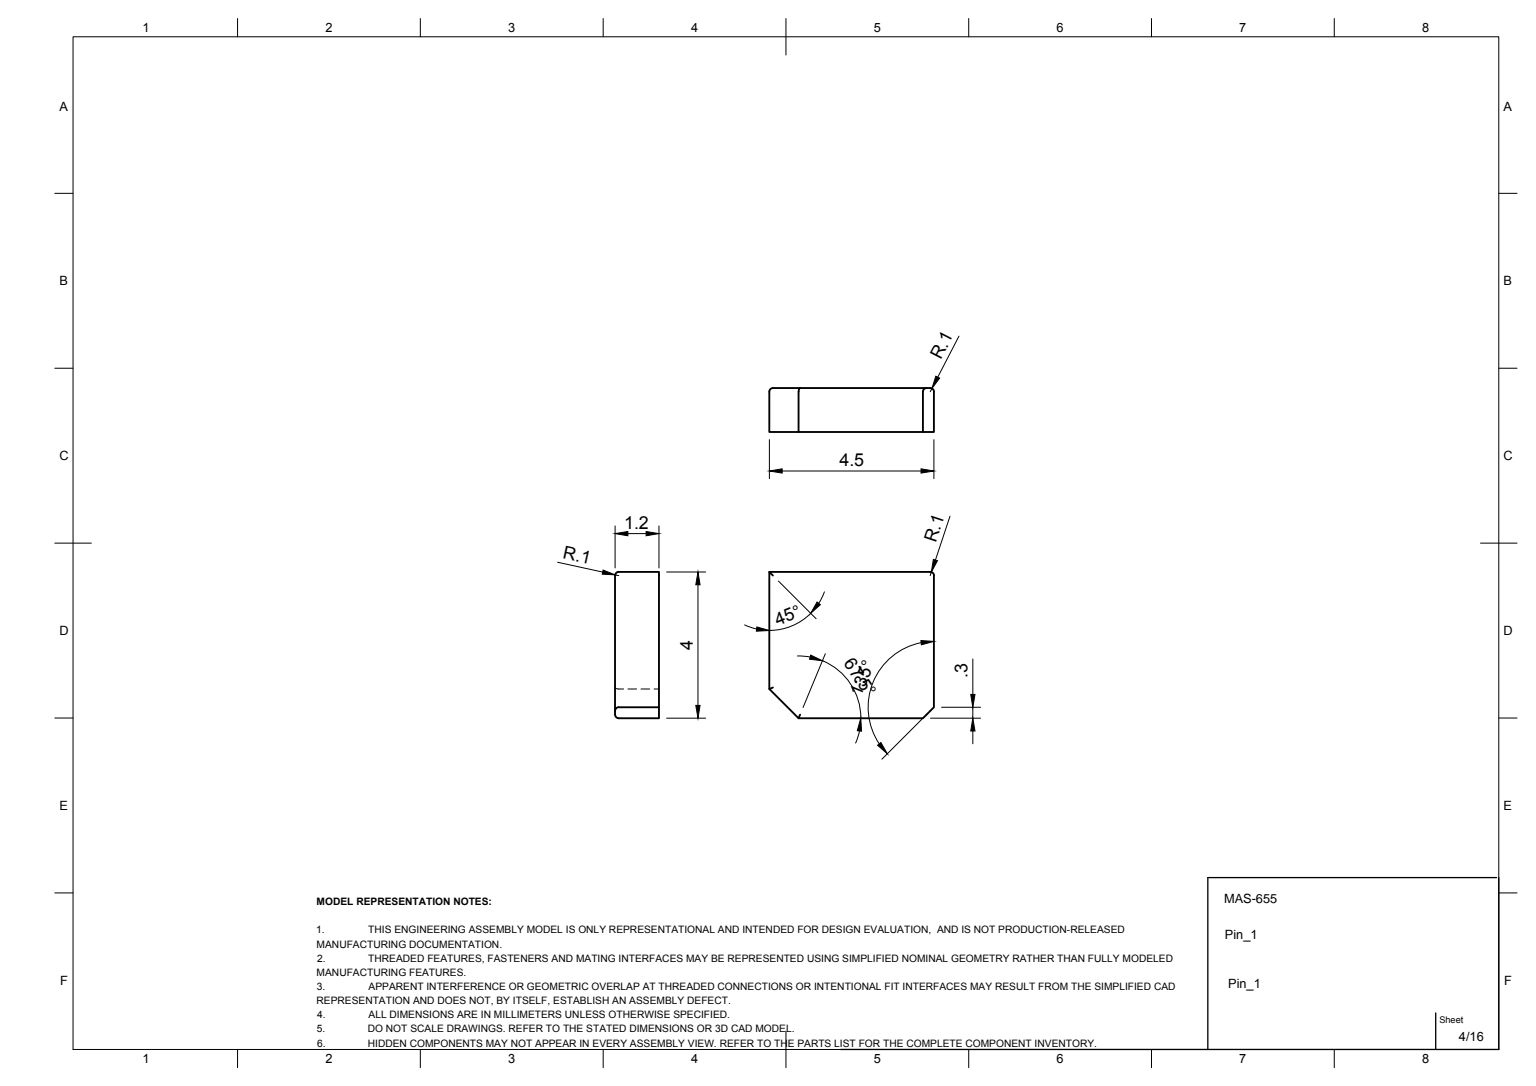
ISO-10303-21;
HEADER;
FILE_DESCRIPTION((''),'2;1');
FILE_NAME('Pin_1.step','2026-10-09T11:34:15-07:00',(''),(''),'','','');
FILE_SCHEMA (('AUTOMOTIVE_DESIGN { 1 0 10303 214 3 1 1 }'));
ENDSEC;
DATA;
#10=MECHANICAL_DESIGN_GEOMETRIC_PRESENTATION_REPRESENTATION('',(#631),#117170);
#264=ELLIPSE('',#51711,0.141421356237302,0.1) ;
#265=ELLIPSE('',#51712,0.108239220029239,0.1) ;
#266=ELLIPSE('',#51714,0.108239220029249,0.1) ;
#267=ELLIPSE('',#51716,0.141421356237297,0.1) ;
#268=ELLIPSE('',#51722,0.141421356237317,0.1) ;
#589=SHAPE_REPRESENTATION_RELATIONSHIP('SRR','None',#117244,#610) ;
#610=ADVANCED_BREP_SHAPE_REPRESENTATION('',(#652),#117152) ;
#631=STYLED_ITEM('',(#117355),#652) ;
#652=MANIFOLD_SOLID_BREP('Body1',#49060) ;
#2192=SPHERICAL_SURFACE('',#51717,0.100000000000016) ;
#2427=PLANE('',#51726) ;
#2428=PLANE('',#51727) ;
#2429=PLANE('',#51728) ;
#2430=PLANE('',#51729) ;
#2431=PLANE('',#51730) ;
#2432=PLANE('',#51731) ;
#2433=PLANE('',#51732) ;
#2434=PLANE('',#51733) ;
#4081=LINE('',#86546,#7295) ;
#4082=LINE('',#86550,#7296) ;
#4083=LINE('',#86554,#7297) ;
#4084=LINE('',#86557,#7298) ;
#4085=LINE('',#86560,#7299) ;
#4086=LINE('',#86563,#7300) ;
#4087=LINE('',#86575,#7301) ;
#4088=LINE('',#86576,#7302) ;
#4089=LINE('',#86581,#7303) ;
#4090=LINE('',#86582,#7304) ;
#4091=LINE('',#86584,#7305) ;
#4092=LINE('',#86585,#7306) ;
#4093=LINE('',#86588,#7307) ;
#4094=LINE('',#86590,#7308) ;
#4095=LINE('',#86591,#7309) ;
#4096=LINE('',#86594,#7310) ;
#4097=LINE('',#86595,#7311) ;
#4098=LINE('',#86596,#7312) ;
#4099=LINE('',#86599,#7313) ;
#4100=LINE('',#86600,#7314) ;
#4101=LINE('',#86603,#7315) ;
#4102=LINE('',#86604,#7316) ;
#4103=LINE('',#86606,#7317) ;
#4104=LINE('',#86608,#7318) ;
#7295=VECTOR('',#60948,10.) ;
#7296=VECTOR('',#60951,10.) ;
#7297=VECTOR('',#60956,10.) ;
#7298=VECTOR('',#60959,10.) ;
#7299=VECTOR('',#60962,10.) ;
#7300=VECTOR('',#60965,10.) ;
#7301=VECTOR('',#60978,10.) ;
#7302=VECTOR('',#60979,10.) ;
#7303=VECTOR('',#60984,10.) ;
#7304=VECTOR('',#60985,10.) ;
#7305=VECTOR('',#60988,10.) ;
#7306=VECTOR('',#60989,10.) ;
#7307=VECTOR('',#60992,10.) ;
#7308=VECTOR('',#60993,10.) ;
#7309=VECTOR('',#60994,10.) ;
#7310=VECTOR('',#60997,10.) ;
#7311=VECTOR('',#60998,10.) ;
#7312=VECTOR('',#60999,10.) ;
#7313=VECTOR('',#61002,10.) ;
#7314=VECTOR('',#61003,10.) ;
#7315=VECTOR('',#61006,10.) ;
#7316=VECTOR('',#61007,10.) ;
#7317=VECTOR('',#61010,10.) ;
#7318=VECTOR('',#61013,10.) ;
#9933=CYLINDRICAL_SURFACE('',#51710,0.1) ;
#9934=CYLINDRICAL_SURFACE('',#51713,0.1) ;
#9935=CYLINDRICAL_SURFACE('',#51715,0.1) ;
#9936=CYLINDRICAL_SURFACE('',#51721,0.1) ;
#9937=CYLINDRICAL_SURFACE('',#51723,0.1) ;
#9938=CYLINDRICAL_SURFACE('',#51725,0.1) ;
#11961=FACE_OUTER_BOUND('',#15105,.T.) ;
#11962=FACE_OUTER_BOUND('',#15106,.T.) ;
#11963=FACE_OUTER_BOUND('',#15107,.T.) ;
#11964=FACE_OUTER_BOUND('',#15108,.T.) ;
#11965=FACE_OUTER_BOUND('',#15109,.T.) ;
#11966=FACE_OUTER_BOUND('',#15110,.T.) ;
#11967=FACE_OUTER_BOUND('',#15111,.T.) ;
#11968=FACE_OUTER_BOUND('',#15112,.T.) ;
#11969=FACE_OUTER_BOUND('',#15113,.T.) ;
#11970=FACE_OUTER_BOUND('',#15114,.T.) ;
#11971=FACE_OUTER_BOUND('',#15115,.T.) ;
#11972=FACE_OUTER_BOUND('',#15116,.T.) ;
#11973=FACE_OUTER_BOUND('',#15117,.T.) ;
#11974=FACE_OUTER_BOUND('',#15118,.T.) ;
#11975=FACE_OUTER_BOUND('',#15119,.T.) ;
#15105=EDGE_LOOP('',(#36600,#36601,#36602,#36603)) ;
#15106=EDGE_LOOP('',(#36604,#36605,#36606,#36607)) ;
#15107=EDGE_LOOP('',(#36608,#36609,#36610,#36611)) ;
#15108=EDGE_LOOP('',(#36612,#36613,#36614)) ;
#15109=EDGE_LOOP('',(#36615,#36616,#36617,#36618)) ;
#15110=EDGE_LOOP('',(#36619,#36620,#36621,#36622)) ;
#15111=EDGE_LOOP('',(#36623,#36624,#36625,#36626)) ;
#15112=EDGE_LOOP('',(#36627,#36628,#36629,#36630)) ;
#15113=EDGE_LOOP('',(#36631,#36632,#36633,#36634,#36635,#36636)) ;
#15114=EDGE_LOOP('',(#36637,#36638,#36639,#36640)) ;
#15115=EDGE_LOOP('',(#36641,#36642,#36643,#36644)) ;
#15116=EDGE_LOOP('',(#36645,#36646,#36647,#36648)) ;
#15117=EDGE_LOOP('',(#36649,#36650,#36651,#36652)) ;
#15118=EDGE_LOOP('',(#36653,#36654,#36655,#36656,#36657,#36658,#36659)) ;
#15119=EDGE_LOOP('',(#36660,#36661,#36662,#36663,#36664,#36665)) ;
#18274=CIRCLE('',#51718,0.0999999999999979) ;
#18275=CIRCLE('',#51719,0.100000000000016) ;
#18276=CIRCLE('',#51720,0.0999999999999979) ;
#18277=CIRCLE('',#51724,0.1) ;
#21170=VERTEX_POINT('',#86544) ;
#21171=VERTEX_POINT('',#86545) ;
#21172=VERTEX_POINT('',#86547) ;
#21173=VERTEX_POINT('',#86549) ;
#21174=VERTEX_POINT('',#86553) ;
#21175=VERTEX_POINT('',#86555) ;
#21176=VERTEX_POINT('',#86559) ;
#21177=VERTEX_POINT('',#86561) ;
#21178=VERTEX_POINT('',#86565) ;
#21179=VERTEX_POINT('',#86566) ;
#21180=VERTEX_POINT('',#86568) ;
#21181=VERTEX_POINT('',#86572) ;
#21182=VERTEX_POINT('',#86573) ;
#21183=VERTEX_POINT('',#86578) ;
#21184=VERTEX_POINT('',#86579) ;
#21185=VERTEX_POINT('',#86587) ;
#21186=VERTEX_POINT('',#86589) ;
#21187=VERTEX_POINT('',#86593) ;
#21188=VERTEX_POINT('',#86598) ;
#21189=VERTEX_POINT('',#86602) ;
#26578=EDGE_CURVE('',#21170,#21171,#4081,.T.) ;
#26579=EDGE_CURVE('',#21171,#21172,#264,.T.) ;
#26580=EDGE_CURVE('',#21172,#21173,#4082,.T.) ;
#26581=EDGE_CURVE('',#21173,#21170,#265,.T.) ;
#26582=EDGE_CURVE('',#21173,#21174,#4083,.T.) ;
#26583=EDGE_CURVE('',#21174,#21175,#266,.T.) ;
#26584=EDGE_CURVE('',#21175,#21170,#4084,.T.) ;
#26585=EDGE_CURVE('',#21174,#21176,#4085,.T.) ;
#26586=EDGE_CURVE('',#21176,#21177,#267,.T.) ;
#26587=EDGE_CURVE('',#21177,#21175,#4086,.T.) ;
#26588=EDGE_CURVE('',#21178,#21179,#18274,.F.) ;
#26589=EDGE_CURVE('',#21180,#21178,#18275,.F.) ;
#26590=EDGE_CURVE('',#21179,#21180,#18276,.F.) ;
#26591=EDGE_CURVE('',#21181,#21182,#268,.T.) ;
#26592=EDGE_CURVE('',#21182,#21180,#4087,.T.) ;
#26593=EDGE_CURVE('',#21178,#21181,#4088,.T.) ;
#26594=EDGE_CURVE('',#21183,#21184,#18277,.T.) ;
#26595=EDGE_CURVE('',#21184,#21179,#4089,.T.) ;
#26596=EDGE_CURVE('',#21180,#21183,#4090,.T.) ;
#26597=EDGE_CURVE('',#21176,#21178,#4091,.T.) ;
#26598=EDGE_CURVE('',#21179,#21177,#4092,.T.) ;
#26599=EDGE_CURVE('',#21170,#21185,#4093,.T.) ;
#26600=EDGE_CURVE('',#21186,#21185,#4094,.T.) ;
#26601=EDGE_CURVE('',#21171,#21186,#4095,.T.) ;
#26602=EDGE_CURVE('',#21187,#21186,#4096,.T.) ;
#26603=EDGE_CURVE('',#21182,#21187,#4097,.T.) ;
#26604=EDGE_CURVE('',#21172,#21181,#4098,.T.) ;
#26605=EDGE_CURVE('',#21175,#21188,#4099,.T.) ;
#26606=EDGE_CURVE('',#21185,#21188,#4100,.T.) ;
#26607=EDGE_CURVE('',#21177,#21189,#4101,.T.) ;
#26608=EDGE_CURVE('',#21188,#21189,#4102,.T.) ;
#26609=EDGE_CURVE('',#21189,#21184,#4103,.T.) ;
#26610=EDGE_CURVE('',#21183,#21187,#4104,.T.) ;
#36600=ORIENTED_EDGE('',*,*,#26578,.T.) ;
#36601=ORIENTED_EDGE('',*,*,#26579,.T.) ;
#36602=ORIENTED_EDGE('',*,*,#26580,.T.) ;
#36603=ORIENTED_EDGE('',*,*,#26581,.T.) ;
#36604=ORIENTED_EDGE('',*,*,#26582,.T.) ;
#36605=ORIENTED_EDGE('',*,*,#26583,.T.) ;
#36606=ORIENTED_EDGE('',*,*,#26584,.T.) ;
#36607=ORIENTED_EDGE('',*,*,#26581,.F.) ;
#36608=ORIENTED_EDGE('',*,*,#26585,.T.) ;
#36609=ORIENTED_EDGE('',*,*,#26586,.T.) ;
#36610=ORIENTED_EDGE('',*,*,#26587,.T.) ;
#36611=ORIENTED_EDGE('',*,*,#26583,.F.) ;
#36612=ORIENTED_EDGE('',*,*,#26588,.F.) ;
#36613=ORIENTED_EDGE('',*,*,#26589,.F.) ;
#36614=ORIENTED_EDGE('',*,*,#26590,.F.) ;
#36615=ORIENTED_EDGE('',*,*,#26591,.T.) ;
#36616=ORIENTED_EDGE('',*,*,#26592,.T.) ;
#36617=ORIENTED_EDGE('',*,*,#26589,.T.) ;
#36618=ORIENTED_EDGE('',*,*,#26593,.T.) ;
#36619=ORIENTED_EDGE('',*,*,#26594,.T.) ;
#36620=ORIENTED_EDGE('',*,*,#26595,.T.) ;
#36621=ORIENTED_EDGE('',*,*,#26590,.T.) ;
#36622=ORIENTED_EDGE('',*,*,#26596,.T.) ;
#36623=ORIENTED_EDGE('',*,*,#26597,.T.) ;
#36624=ORIENTED_EDGE('',*,*,#26588,.T.) ;
#36625=ORIENTED_EDGE('',*,*,#26598,.T.) ;
#36626=ORIENTED_EDGE('',*,*,#26586,.F.) ;
#36627=ORIENTED_EDGE('',*,*,#26578,.F.) ;
#36628=ORIENTED_EDGE('',*,*,#26599,.T.) ;
#36629=ORIENTED_EDGE('',*,*,#26600,.F.) ;
#36630=ORIENTED_EDGE('',*,*,#26601,.F.) ;
#36631=ORIENTED_EDGE('',*,*,#26579,.F.) ;
#36632=ORIENTED_EDGE('',*,*,#26601,.T.) ;
#36633=ORIENTED_EDGE('',*,*,#26602,.F.) ;
#36634=ORIENTED_EDGE('',*,*,#26603,.F.) ;
#36635=ORIENTED_EDGE('',*,*,#26591,.F.) ;
#36636=ORIENTED_EDGE('',*,*,#26604,.F.) ;
#36637=ORIENTED_EDGE('',*,*,#26584,.F.) ;
#36638=ORIENTED_EDGE('',*,*,#26605,.T.) ;
#36639=ORIENTED_EDGE('',*,*,#26606,.F.) ;
#36640=ORIENTED_EDGE('',*,*,#26599,.F.) ;
#36641=ORIENTED_EDGE('',*,*,#26587,.F.) ;
#36642=ORIENTED_EDGE('',*,*,#26607,.T.) ;
#36643=ORIENTED_EDGE('',*,*,#26608,.F.) ;
#36644=ORIENTED_EDGE('',*,*,#26605,.F.) ;
#36645=ORIENTED_EDGE('',*,*,#26598,.F.) ;
#36646=ORIENTED_EDGE('',*,*,#26595,.F.) ;
#36647=ORIENTED_EDGE('',*,*,#26609,.F.) ;
#36648=ORIENTED_EDGE('',*,*,#26607,.F.) ;
#36649=ORIENTED_EDGE('',*,*,#26592,.F.) ;
#36650=ORIENTED_EDGE('',*,*,#26603,.T.) ;
#36651=ORIENTED_EDGE('',*,*,#26610,.F.) ;
#36652=ORIENTED_EDGE('',*,*,#26596,.F.) ;
#36653=ORIENTED_EDGE('',*,*,#26594,.F.) ;
#36654=ORIENTED_EDGE('',*,*,#26610,.T.) ;
#36655=ORIENTED_EDGE('',*,*,#26602,.T.) ;
#36656=ORIENTED_EDGE('',*,*,#26600,.T.) ;
#36657=ORIENTED_EDGE('',*,*,#26606,.T.) ;
#36658=ORIENTED_EDGE('',*,*,#26608,.T.) ;
#36659=ORIENTED_EDGE('',*,*,#26609,.T.) ;
#36660=ORIENTED_EDGE('',*,*,#26580,.F.) ;
#36661=ORIENTED_EDGE('',*,*,#26604,.T.) ;
#36662=ORIENTED_EDGE('',*,*,#26593,.F.) ;
#36663=ORIENTED_EDGE('',*,*,#26597,.F.) ;
#36664=ORIENTED_EDGE('',*,*,#26585,.F.) ;
#36665=ORIENTED_EDGE('',*,*,#26582,.F.) ;
#47179=ADVANCED_FACE('',(#11961),#9933,.T.) ;
#47180=ADVANCED_FACE('',(#11962),#9934,.T.) ;
#47181=ADVANCED_FACE('',(#11963),#9935,.T.) ;
#47182=ADVANCED_FACE('',(#11964),#2192,.T.) ;
#47183=ADVANCED_FACE('',(#11965),#9936,.T.) ;
#47184=ADVANCED_FACE('',(#11966),#9937,.T.) ;
#47185=ADVANCED_FACE('',(#11967),#9938,.T.) ;
#47186=ADVANCED_FACE('',(#11968),#2427,.T.) ;
#47187=ADVANCED_FACE('',(#11969),#2428,.T.) ;
#47188=ADVANCED_FACE('',(#11970),#2429,.T.) ;
#47189=ADVANCED_FACE('',(#11971),#2430,.T.) ;
#47190=ADVANCED_FACE('',(#11972),#2431,.T.) ;
#47191=ADVANCED_FACE('',(#11973),#2432,.T.) ;
#47192=ADVANCED_FACE('',(#11974),#2433,.T.) ;
#47193=ADVANCED_FACE('',(#11975),#2434,.F.) ;
#49060=CLOSED_SHELL('',(#47179,#47180,#47181,#47182,#47183,#47184,#47185,
#47186,#47187,#47188,#47189,#47190,#47191,#47192,#47193)) ;
#51709=AXIS2_PLACEMENT_3D('',#86542,#60944,#60945) ;
#51710=AXIS2_PLACEMENT_3D('',#86543,#60946,#60947) ;
#51711=AXIS2_PLACEMENT_3D('',#86548,#60949,#60950) ;
#51712=AXIS2_PLACEMENT_3D('',#86551,#60952,#60953) ;
#51713=AXIS2_PLACEMENT_3D('',#86552,#60954,#60955) ;
#51714=AXIS2_PLACEMENT_3D('',#86556,#60957,#60958) ;
#51715=AXIS2_PLACEMENT_3D('',#86558,#60960,#60961) ;
#51716=AXIS2_PLACEMENT_3D('',#86562,#60963,#60964) ;
#51717=AXIS2_PLACEMENT_3D('',#86564,#60966,#60967) ;
#51718=AXIS2_PLACEMENT_3D('',#86567,#60968,#60969) ;
#51719=AXIS2_PLACEMENT_3D('',#86569,#60970,#60971) ;
#51720=AXIS2_PLACEMENT_3D('',#86570,#60972,#60973) ;
#51721=AXIS2_PLACEMENT_3D('',#86571,#60974,#60975) ;
#51722=AXIS2_PLACEMENT_3D('',#86574,#60976,#60977) ;
#51723=AXIS2_PLACEMENT_3D('',#86577,#60980,#60981) ;
#51724=AXIS2_PLACEMENT_3D('',#86580,#60982,#60983) ;
#51725=AXIS2_PLACEMENT_3D('',#86583,#60986,#60987) ;
#51726=AXIS2_PLACEMENT_3D('',#86586,#60990,#60991) ;
#51727=AXIS2_PLACEMENT_3D('',#86592,#60995,#60996) ;
#51728=AXIS2_PLACEMENT_3D('',#86597,#61000,#61001) ;
#51729=AXIS2_PLACEMENT_3D('',#86601,#61004,#61005) ;
#51730=AXIS2_PLACEMENT_3D('',#86605,#61008,#61009) ;
#51731=AXIS2_PLACEMENT_3D('',#86607,#61011,#61012) ;
#51732=AXIS2_PLACEMENT_3D('',#86609,#61014,#61015) ;
#51733=AXIS2_PLACEMENT_3D('',#86610,#61016,#61017) ;
#60944=DIRECTION('axis',(0.,0.,1.)) ;
#60945=DIRECTION('refdir',(1.,0.,0.)) ;
#60946=DIRECTION('center_axis',(-5.22457893941245E-15,-1.,-1.37458674256137E-32)) ;
#60947=DIRECTION('ref_axis',(-0.707106781186548,3.69433519690296E-15,0.707106781186548)) ;
#60948=DIRECTION('',(-5.22457893941245E-15,-1.,-1.37458674256137E-32)) ;
#60949=DIRECTION('center_axis',(0.707106781186512,0.707106781186583,0.)) ;
#60950=DIRECTION('ref_axis',(-0.707106781186583,0.707106781186512,6.13317366673383E-17)) ;
#60951=DIRECTION('',(5.22457893941245E-15,1.,1.37458674256137E-32)) ;
#60952=DIRECTION('center_axis',(-0.382683432365083,-0.92387953251129,0.)) ;
#60953=DIRECTION('ref_axis',(-0.92387953251129,0.382683432365083,3.59196825968159E-32)) ;
#60954=DIRECTION('center_axis',(-0.707106781186555,-0.70710678118654,-1.78455441078682E-18)) ;
#60955=DIRECTION('ref_axis',(-0.499999999999962,0.499999999999972,0.707106781186594)) ;
#60956=DIRECTION('',(0.707106781186555,0.70710678118654,1.78455441078682E-18)) ;
#60957=DIRECTION('center_axis',(-0.923879532511372,-0.382683432364885,0.)) ;
#60958=DIRECTION('ref_axis',(-0.382683432364885,0.923879532511372,4.66326540387932E-18)) ;
#60959=DIRECTION('',(-0.707106781186555,-0.70710678118654,-1.78455441078682E-18)) ;
#60960=DIRECTION('center_axis',(-1.,0.,-2.52374105052742E-18)) ;
#60961=DIRECTION('ref_axis',(-1.78455441078696E-18,0.707106781186485,0.70710678118661)) ;
#60962=DIRECTION('',(1.,0.,2.52374105052742E-18)) ;
#60963=DIRECTION('center_axis',(-0.70710678118661,0.707106781186485,0.)) ;
#60964=DIRECTION('ref_axis',(0.707106781186485,0.70710678118661,3.56910882157392E-18)) ;
#60965=DIRECTION('',(-1.,0.,-2.52374105052742E-18)) ;
#60966=DIRECTION('center_axis',(-0.816496580927762,-0.40824829046381,0.408248290463845)) ;
#60967=DIRECTION('ref_axis',(0.577350269189543,-0.577350269189685,0.577350269189649)) ;
#60968=DIRECTION('center_axis',(0.,-1.,0.)) ;
#60969=DIRECTION('ref_axis',(0.,0.,1.)) ;
#60970=DIRECTION('center_axis',(1.,0.,0.)) ;
#60971=DIRECTION('ref_axis',(0.,-1.,0.)) ;
#60972=DIRECTION('center_axis',(0.,0.,1.)) ;
#60973=DIRECTION('ref_axis',(1.,0.,0.)) ;
#60974=DIRECTION('center_axis',(1.,0.,2.52374105052742E-18)) ;
#60975=DIRECTION('ref_axis',(-1.78455441078632E-18,-0.707106781186736,0.707106781186359)) ;
#60976=DIRECTION('center_axis',(0.707106781186512,0.707106781186583,0.)) ;
#60977=DIRECTION('ref_axis',(0.707106781186583,-0.707106781186512,-1.83995210001996E-16)) ;
#60978=DIRECTION('',(1.,0.,2.52374105052742E-18)) ;
#60979=DIRECTION('',(-1.,0.,-2.52374105052742E-18)) ;
#60980=DIRECTION('center_axis',(0.,0.,-1.)) ;
#60981=DIRECTION('ref_axis',(0.707106781186359,-0.707106781186736,0.)) ;
#60982=DIRECTION('center_axis',(0.,0.,1.)) ;
#60983=DIRECTION('ref_axis',(0.707106781186359,-0.707106781186736,0.)) ;
#60984=DIRECTION('',(0.,0.,1.)) ;
#60985=DIRECTION('',(0.,0.,-1.)) ;
#60986=DIRECTION('center_axis',(-1.41426179436738E-51,1.,5.60383084497445E-34)) ;
#60987=DIRECTION('ref_axis',(0.707106781186548,-3.96250679110377E-34,0.707106781186548)) ;
#60988=DIRECTION('',(1.41426179436738E-51,-1.,-5.60383084497445E-34)) ;
#60989=DIRECTION('',(-1.41426179436738E-51,1.,5.60383084497445E-34)) ;
#60990=DIRECTION('center_axis',(-1.,5.22457893941245E-15,0.)) ;
#60991=DIRECTION('ref_axis',(5.22457893941245E-15,1.,1.37458674256137E-32)) ;
#60992=DIRECTION('',(0.,0.,-1.)) ;
#60993=DIRECTION('',(5.22457893941245E-15,1.,1.37458674256137E-32)) ;
#60994=DIRECTION('',(0.,0.,-1.)) ;
#60995=DIRECTION('center_axis',(-0.707106781186512,-0.707106781186583,0.)) ;
#60996=DIRECTION('ref_axis',(-0.707106781186583,0.707106781186512,-1.78455441078689E-18)) ;
#60997=DIRECTION('',(-0.707106781186583,0.707106781186512,-1.78455441078689E-18)) ;
#60998=DIRECTION('',(0.,0.,-1.)) ;
#60999=DIRECTION('',(0.707106781186583,-0.707106781186512,1.78455441078689E-18)) ;
#61000=DIRECTION('center_axis',(-0.70710678118654,0.707106781186555,0.)) ;
#61001=DIRECTION('ref_axis',(0.707106781186555,0.70710678118654,1.78455441078682E-18)) ;
#61002=DIRECTION('',(0.,0.,-1.)) ;
#61003=DIRECTION('',(0.707106781186555,0.70710678118654,1.78455441078682E-18)) ;
#61004=DIRECTION('center_axis',(0.,1.,0.)) ;
#61005=DIRECTION('ref_axis',(1.,0.,2.52374105052742E-18)) ;
#61006=DIRECTION('',(0.,0.,-1.)) ;
#61007=DIRECTION('',(1.,0.,2.52374105052742E-18)) ;
#61008=DIRECTION('center_axis',(1.,1.41426179436738E-51,0.)) ;
#61009=DIRECTION('ref_axis',(1.41426179436738E-51,-1.,-5.60383084497445E-34)) ;
#61010=DIRECTION('',(1.41426179436738E-51,-1.,-5.60383084497445E-34)) ;
#61011=DIRECTION('center_axis',(0.,-1.,0.)) ;
#61012=DIRECTION('ref_axis',(-1.,0.,-2.52374105052742E-18)) ;
#61013=DIRECTION('',(-1.,0.,-2.52374105052742E-18)) ;
#61014=DIRECTION('center_axis',(0.,0.,-1.)) ;
#61015=DIRECTION('ref_axis',(-1.,0.,0.)) ;
#61016=DIRECTION('center_axis',(2.52374105052742E-18,5.60383084497445E-34,
-1.)) ;
#61017=DIRECTION('ref_axis',(1.,3.40207761657885E-68,2.52374105052742E-18)) ;
#86542=CARTESIAN_POINT('',(0.,0.,0.)) ;
#86543=CARTESIAN_POINT('Origin',(75.3,227.275,30.6213203435596)) ;
#86544=CARTESIAN_POINT('',(75.2,229.7,30.6213203435596)) ;
#86545=CARTESIAN_POINT('',(75.1999999999999,226.3,30.6213203435596)) ;
#86546=CARTESIAN_POINT('',(75.1999999999999,227.275,30.6213203435596)) ;
#86547=CARTESIAN_POINT('',(75.2999999999999,226.2,30.7213203435596)) ;
#86548=CARTESIAN_POINT('Origin',(75.2999999999999,226.2,30.6213203435596)) ;
#86549=CARTESIAN_POINT('',(75.3,229.658578643763,30.7213203435596)) ;
#86550=CARTESIAN_POINT('',(75.3,227.275,30.7213203435596)) ;
#86551=CARTESIAN_POINT('Origin',(75.3,229.658578643763,30.6213203435596)) ;
#86552=CARTESIAN_POINT('Origin',(75.4082106781188,229.766789321882,30.6213203435596)) ;
#86553=CARTESIAN_POINT('',(76.0414213562373,230.4,30.7213203435596)) ;
#86554=CARTESIAN_POINT('',(75.4082106781188,229.766789321882,30.7213203435596)) ;
#86555=CARTESIAN_POINT('',(76.,230.5,30.6213203435596)) ;
#86556=CARTESIAN_POINT('Origin',(76.0414213562373,230.4,30.6213203435596)) ;
#86557=CARTESIAN_POINT('',(75.3375000000001,229.8375,30.6213203435596)) ;
#86558=CARTESIAN_POINT('Origin',(76.6,230.4,30.6213203435596)) ;
#86559=CARTESIAN_POINT('',(79.1,230.4,30.7213203435596)) ;
#86560=CARTESIAN_POINT('',(76.6,230.4,30.7213203435596)) ;
#86561=CARTESIAN_POINT('',(79.2,230.5,30.6213203435596)) ;
#86562=CARTESIAN_POINT('Origin',(79.1,230.4,30.6213203435596)) ;
#86563=CARTESIAN_POINT('',(76.6,230.5,30.6213203435596)) ;
#86564=CARTESIAN_POINT('Origin',(79.1,226.100000000001,30.6213203435596)) ;
#86565=CARTESIAN_POINT('',(79.1,226.100000000001,30.7213203435596)) ;
#86566=CARTESIAN_POINT('',(79.2,226.100000000001,30.6213203435596)) ;
#86567=CARTESIAN_POINT('Origin',(79.1,226.100000000001,30.6213203435596)) ;
#86568=CARTESIAN_POINT('',(79.1,226.000000000001,30.6213203435596)) ;
#86569=CARTESIAN_POINT('Origin',(79.1,226.100000000001,30.6213203435596)) ;
#86570=CARTESIAN_POINT('Origin',(79.1,226.100000000001,30.6213203435596)) ;
#86571=CARTESIAN_POINT('Origin',(78.2,226.100000000001,30.6213203435596)) ;
#86572=CARTESIAN_POINT('',(75.3999999999987,226.100000000001,30.7213203435596)) ;
#86573=CARTESIAN_POINT('',(75.4999999999987,226.000000000001,30.6213203435596)) ;
#86574=CARTESIAN_POINT('Origin',(75.3999999999987,226.100000000001,30.6213203435596)) ;
#86575=CARTESIAN_POINT('',(78.2,226.000000000001,30.6213203435596)) ;
#86576=CARTESIAN_POINT('',(78.2,226.100000000001,30.7213203435596)) ;
#86577=CARTESIAN_POINT('Origin',(79.1,226.100000000001,30.7213203435596)) ;
#86578=CARTESIAN_POINT('',(79.1,226.000000000001,29.5213203435596)) ;
#86579=CARTESIAN_POINT('',(79.2,226.100000000001,29.5213203435596)) ;
#86580=CARTESIAN_POINT('Origin',(79.1,226.100000000001,29.5213203435596)) ;
#86581=CARTESIAN_POINT('',(79.2,226.100000000001,30.7213203435596)) ;
#86582=CARTESIAN_POINT('',(79.1,226.000000000001,30.7213203435596)) ;
#86583=CARTESIAN_POINT('Origin',(79.1,229.375,30.6213203435596)) ;
#86584=CARTESIAN_POINT('',(79.1,229.375,30.7213203435596)) ;
#86585=CARTESIAN_POINT('',(79.2,229.375,30.6213203435596)) ;
#86586=CARTESIAN_POINT('Origin',(75.1999999999999,226.3,30.7213203435596)) ;
#86587=CARTESIAN_POINT('',(75.2,229.7,29.5213203435596)) ;
#86588=CARTESIAN_POINT('',(75.2,229.7,30.7213203435596)) ;
#86589=CARTESIAN_POINT('',(75.1999999999999,226.3,29.5213203435596)) ;
#86590=CARTESIAN_POINT('',(75.2,229.7,29.5213203435596)) ;
#86591=CARTESIAN_POINT('',(75.1999999999999,226.3,30.7213203435596)) ;
#86592=CARTESIAN_POINT('Origin',(75.4999999999987,226.000000000001,30.7213203435596)) ;
#86593=CARTESIAN_POINT('',(75.4999999999987,226.000000000001,29.5213203435596)) ;
#86594=CARTESIAN_POINT('',(75.1999999999999,226.3,29.5213203435596)) ;
#86595=CARTESIAN_POINT('',(75.4999999999987,226.000000000001,30.7213203435596)) ;
#86596=CARTESIAN_POINT('',(75.1999999999999,226.3,30.7213203435596)) ;
#86597=CARTESIAN_POINT('Origin',(75.2,229.7,30.7213203435596)) ;
#86598=CARTESIAN_POINT('',(76.,230.5,29.5213203435596)) ;
#86599=CARTESIAN_POINT('',(76.,230.5,30.7213203435596)) ;
#86600=CARTESIAN_POINT('',(76.,230.5,29.5213203435596)) ;
#86601=CARTESIAN_POINT('Origin',(76.,230.5,30.7213203435596)) ;
#86602=CARTESIAN_POINT('',(79.2,230.5,29.5213203435596)) ;
#86603=CARTESIAN_POINT('',(79.2,230.5,30.7213203435596)) ;
#86604=CARTESIAN_POINT('',(80.2,230.5,29.5213203435596)) ;
#86605=CARTESIAN_POINT('Origin',(79.2,230.5,30.7213203435596)) ;
#86606=CARTESIAN_POINT('',(79.2,226.000000000001,29.5213203435596)) ;
#86607=CARTESIAN_POINT('Origin',(79.2,226.000000000001,30.7213203435596)) ;
#86608=CARTESIAN_POINT('',(74.7,226.000000000001,29.5213203435596)) ;
#86609=CARTESIAN_POINT('Origin',(77.2,228.250000000001,29.5213203435596)) ;
#86610=CARTESIAN_POINT('Origin',(77.2,228.250000000001,30.7213203435596)) ;
#117129=UNCERTAINTY_MEASURE_WITH_UNIT(LENGTH_MEASURE(0.01),#117171,
'DISTANCE_ACCURACY_VALUE',
'Maximum model space distance between geometric entities at asserted c
onnectivities') ;
#117147=UNCERTAINTY_MEASURE_WITH_UNIT(LENGTH_MEASURE(0.01),#117171,
'DISTANCE_ACCURACY_VALUE',
'Maximum model space distance between geometric entities at asserted c
onnectivities') ;
#117152=(
GEOMETRIC_REPRESENTATION_CONTEXT(3)
GLOBAL_UNCERTAINTY_ASSIGNED_CONTEXT((#117129))
GLOBAL_UNIT_ASSIGNED_CONTEXT((#117171,#117173,#117174))
REPRESENTATION_CONTEXT('','3D')
) ;
#117170=(
GEOMETRIC_REPRESENTATION_CONTEXT(3)
GLOBAL_UNCERTAINTY_ASSIGNED_CONTEXT((#117147))
GLOBAL_UNIT_ASSIGNED_CONTEXT((#117171,#117173,#117174))
REPRESENTATION_CONTEXT('','3D')
) ;
#117171=(
LENGTH_UNIT()
NAMED_UNIT(*)
SI_UNIT(.MILLI.,.METRE.)
) ;
#117173=(
NAMED_UNIT(*)
PLANE_ANGLE_UNIT()
SI_UNIT($,.RADIAN.)
) ;
#117174=(
NAMED_UNIT(*)
SI_UNIT($,.STERADIAN.)
SOLID_ANGLE_UNIT()
) ;
#117179=SHAPE_DEFINITION_REPRESENTATION(#117201,#117244) ;
#117201=PRODUCT_DEFINITION_SHAPE('',$,#117267) ;
#117244=SHAPE_REPRESENTATION('',(#51709),#117152) ;
#117262=PRODUCT_DEFINITION_CONTEXT('part definition',#117330,'design') ;
#117267=PRODUCT_DEFINITION('Pin_1','Pin_1',#117289,#117262) ;
#117289=PRODUCT_DEFINITION_FORMATION('',$,#117336) ;
#117330=APPLICATION_CONTEXT(
'Core Data for Automotive Mechanical Design Process') ;
#117331=PRODUCT_CONTEXT('part definition',#117330,'mechanical') ;
#117336=PRODUCT('Pin_1','Pin_1',$,(#117331)) ;
#117355=PRESENTATION_STYLE_ASSIGNMENT((#117357)) ;
#117357=SURFACE_STYLE_USAGE(.BOTH.,#117359) ;
#117359=SURFACE_SIDE_STYLE('',(#117361)) ;
#117361=SURFACE_STYLE_FILL_AREA(#117363) ;
#117363=FILL_AREA_STYLE('Opaque(160,160,160)',(#117365)) ;
#117365=FILL_AREA_STYLE_COLOUR('Opaque(160,160,160)',#117367) ;
#117367=COLOUR_RGB('Opaque(160,160,160)', 0.09019608, 0.27058824, 0.51372549) ;
ENDSEC;
END-ISO-10303-21;
